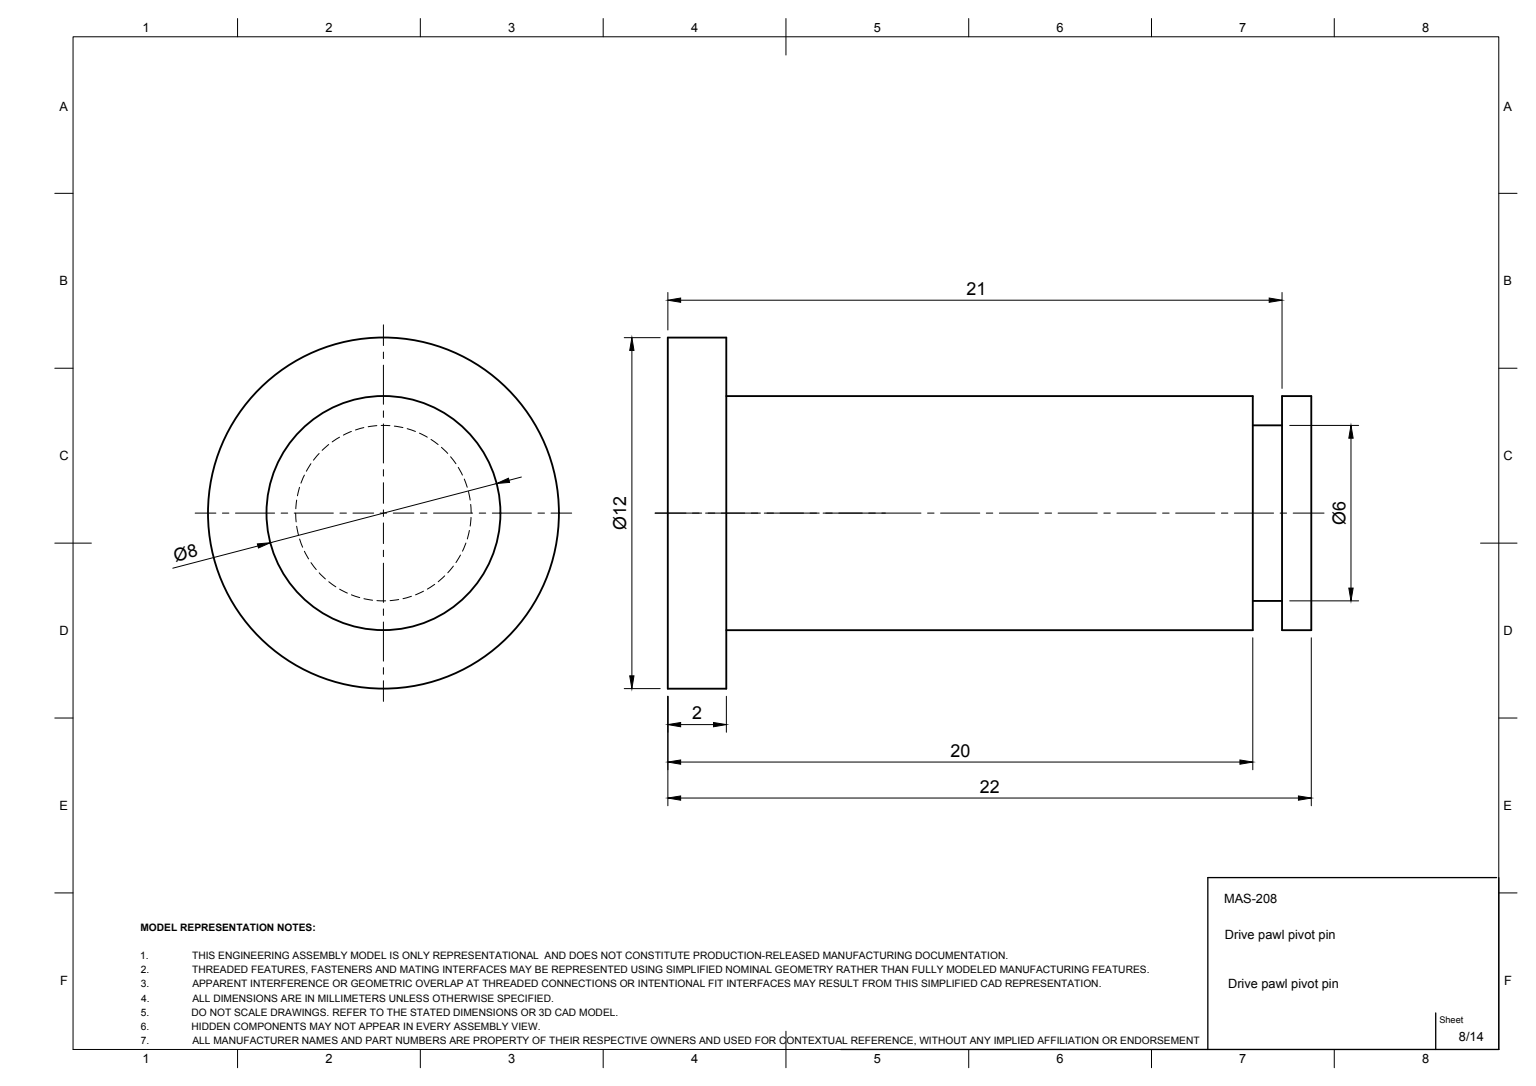
ISO-10303-21;
HEADER;
/* Generated by software containing ST-Developer
 * from STEP Tools, Inc. (www.steptools.com) 
 */

FILE_DESCRIPTION(
/* description */ ('Independent vertical20-tooth ratchet advance with repeated integral-c
ounterweight gravity pawls, swinging drive lever, bronze sleeves and f
ully retained axle stacks.18degpertooth. Native revolutes; geometric c
ycle checking rather than automatic contact/rolling dynamics. Gravity 
closing checked from actual pawl center of mass. Backplate/foot suppor
ts unit. Fits, torque, holding force, wear and life unassigned.'),
/* implementation_level */ '2;1');

FILE_NAME(
/* name */ 'Drive pawl pivot pin.step',
/* time_stamp */ '2026-11-09T06:25:53-08:00',
/* author */ (''),
/* organization */ (''),
/* preprocessor_version */ 'ST-DEVELOPER v20.2',
/* originating_system */ 'Autodesk Translation Framework v15.17.0.0',
/* authorisation */ '');

FILE_SCHEMA (('AUTOMOTIVE_DESIGN { 1 0 10303 214 3 1 1 }'));
ENDSEC;

DATA;
#10=MECHANICAL_DESIGN_GEOMETRIC_PRESENTATION_REPRESENTATION('',(#127),#4643);
#99=SHAPE_REPRESENTATION_RELATIONSHIP('SRR','None',#4704,#113);
#113=ADVANCED_BREP_SHAPE_REPRESENTATION('',(#141),#4633);
#127=STYLED_ITEM('',(#4782),#141);
#141=MANIFOLD_SOLID_BREP('Body1',#2663);
#174=FACE_BOUND('',#559,.T.);
#175=FACE_BOUND('',#561,.T.);
#176=FACE_BOUND('',#564,.T.);
#259=PLANE('',#2946);
#260=PLANE('',#2948);
#261=PLANE('',#2952);
#262=PLANE('',#2957);
#263=PLANE('',#2959);
#385=FACE_OUTER_BOUND('',#557,.T.);
#386=FACE_OUTER_BOUND('',#558,.T.);
#387=FACE_OUTER_BOUND('',#560,.T.);
#388=FACE_OUTER_BOUND('',#562,.T.);
#389=FACE_OUTER_BOUND('',#563,.T.);
#390=FACE_OUTER_BOUND('',#565,.T.);
#391=FACE_OUTER_BOUND('',#566,.T.);
#392=FACE_OUTER_BOUND('',#567,.T.);
#393=FACE_OUTER_BOUND('',#568,.T.);
#557=EDGE_LOOP('',(#2221,#2222,#2223,#2224));
#558=EDGE_LOOP('',(#2225));
#559=EDGE_LOOP('',(#2226));
#560=EDGE_LOOP('',(#2227));
#561=EDGE_LOOP('',(#2228));
#562=EDGE_LOOP('',(#2229,#2230,#2231,#2232));
#563=EDGE_LOOP('',(#2233));
#564=EDGE_LOOP('',(#2234));
#565=EDGE_LOOP('',(#2235,#2236,#2237,#2238));
#566=EDGE_LOOP('',(#2239));
#567=EDGE_LOOP('',(#2240,#2241,#2242,#2243));
#568=EDGE_LOOP('',(#2244));
#825=LINE('',#4308,#1087);
#826=LINE('',#4319,#1088);
#827=LINE('',#4327,#1089);
#828=LINE('',#4331,#1090);
#1087=VECTOR('',#3503,3.);
#1088=VECTOR('',#3518,4.);
#1089=VECTOR('',#3527,6.);
#1090=VECTOR('',#3534,4.);
#1195=CIRCLE('',#2944,3.);
#1196=CIRCLE('',#2945,3.);
#1197=CIRCLE('',#2947,4.);
#1198=CIRCLE('',#2949,4.);
#1199=CIRCLE('',#2951,4.);
#1200=CIRCLE('',#2953,6.);
#1201=CIRCLE('',#2954,4.);
#1202=CIRCLE('',#2956,6.);
#1381=VERTEX_POINT('',#4305);
#1382=VERTEX_POINT('',#4307);
#1383=VERTEX_POINT('',#4311);
#1384=VERTEX_POINT('',#4314);
#1385=VERTEX_POINT('',#4317);
#1386=VERTEX_POINT('',#4321);
#1387=VERTEX_POINT('',#4323);
#1388=VERTEX_POINT('',#4326);
#1675=EDGE_CURVE('',#1381,#1381,#1195,.T.);
#1676=EDGE_CURVE('',#1381,#1382,#825,.T.);
#1677=EDGE_CURVE('',#1382,#1382,#1196,.T.);
#1678=EDGE_CURVE('',#1383,#1383,#1197,.T.);
#1679=EDGE_CURVE('',#1384,#1384,#1198,.T.);
#1680=EDGE_CURVE('',#1385,#1385,#1199,.T.);
#1681=EDGE_CURVE('',#1385,#1384,#826,.T.);
#1682=EDGE_CURVE('',#1386,#1386,#1200,.T.);
#1683=EDGE_CURVE('',#1387,#1387,#1201,.T.);
#1684=EDGE_CURVE('',#1386,#1388,#827,.T.);
#1685=EDGE_CURVE('',#1388,#1388,#1202,.T.);
#1686=EDGE_CURVE('',#1383,#1387,#828,.T.);
#2221=ORIENTED_EDGE('',*,*,#1675,.T.);
#2222=ORIENTED_EDGE('',*,*,#1676,.T.);
#2223=ORIENTED_EDGE('',*,*,#1677,.F.);
#2224=ORIENTED_EDGE('',*,*,#1676,.F.);
#2225=ORIENTED_EDGE('',*,*,#1678,.F.);
#2226=ORIENTED_EDGE('',*,*,#1675,.F.);
#2227=ORIENTED_EDGE('',*,*,#1679,.F.);
#2228=ORIENTED_EDGE('',*,*,#1677,.T.);
#2229=ORIENTED_EDGE('',*,*,#1680,.F.);
#2230=ORIENTED_EDGE('',*,*,#1681,.T.);
#2231=ORIENTED_EDGE('',*,*,#1679,.T.);
#2232=ORIENTED_EDGE('',*,*,#1681,.F.);
#2233=ORIENTED_EDGE('',*,*,#1682,.T.);
#2234=ORIENTED_EDGE('',*,*,#1683,.F.);
#2235=ORIENTED_EDGE('',*,*,#1682,.F.);
#2236=ORIENTED_EDGE('',*,*,#1684,.T.);
#2237=ORIENTED_EDGE('',*,*,#1685,.T.);
#2238=ORIENTED_EDGE('',*,*,#1684,.F.);
#2239=ORIENTED_EDGE('',*,*,#1685,.F.);
#2240=ORIENTED_EDGE('',*,*,#1678,.T.);
#2241=ORIENTED_EDGE('',*,*,#1686,.T.);
#2242=ORIENTED_EDGE('',*,*,#1683,.T.);
#2243=ORIENTED_EDGE('',*,*,#1686,.F.);
#2244=ORIENTED_EDGE('',*,*,#1680,.T.);
#2487=CYLINDRICAL_SURFACE('',#2943,3.);
#2488=CYLINDRICAL_SURFACE('',#2950,4.);
#2489=CYLINDRICAL_SURFACE('',#2955,6.);
#2490=CYLINDRICAL_SURFACE('',#2958,4.);
#2591=ADVANCED_FACE('',(#385),#2487,.T.);
#2592=ADVANCED_FACE('',(#386,#174),#259,.F.);
#2593=ADVANCED_FACE('',(#387,#175),#260,.F.);
#2594=ADVANCED_FACE('',(#388),#2488,.T.);
#2595=ADVANCED_FACE('',(#389,#176),#261,.T.);
#2596=ADVANCED_FACE('',(#390),#2489,.T.);
#2597=ADVANCED_FACE('',(#391),#262,.F.);
#2598=ADVANCED_FACE('',(#392),#2490,.T.);
#2599=ADVANCED_FACE('',(#393),#263,.T.);
#2663=CLOSED_SHELL('',(#2591,#2592,#2593,#2594,#2595,#2596,#2597,#2598,
#2599));
#2942=AXIS2_PLACEMENT_3D('',#4303,#3497,#3498);
#2943=AXIS2_PLACEMENT_3D('',#4304,#3499,#3500);
#2944=AXIS2_PLACEMENT_3D('',#4306,#3501,#3502);
#2945=AXIS2_PLACEMENT_3D('',#4309,#3504,#3505);
#2946=AXIS2_PLACEMENT_3D('',#4310,#3506,#3507);
#2947=AXIS2_PLACEMENT_3D('',#4312,#3508,#3509);
#2948=AXIS2_PLACEMENT_3D('',#4313,#3510,#3511);
#2949=AXIS2_PLACEMENT_3D('',#4315,#3512,#3513);
#2950=AXIS2_PLACEMENT_3D('',#4316,#3514,#3515);
#2951=AXIS2_PLACEMENT_3D('',#4318,#3516,#3517);
#2952=AXIS2_PLACEMENT_3D('',#4320,#3519,#3520);
#2953=AXIS2_PLACEMENT_3D('',#4322,#3521,#3522);
#2954=AXIS2_PLACEMENT_3D('',#4324,#3523,#3524);
#2955=AXIS2_PLACEMENT_3D('',#4325,#3525,#3526);
#2956=AXIS2_PLACEMENT_3D('',#4328,#3528,#3529);
#2957=AXIS2_PLACEMENT_3D('',#4329,#3530,#3531);
#2958=AXIS2_PLACEMENT_3D('',#4330,#3532,#3533);
#2959=AXIS2_PLACEMENT_3D('',#4332,#3535,#3536);
#3497=DIRECTION('axis',(0.,0.,1.));
#3498=DIRECTION('refdir',(1.,0.,0.));
#3499=DIRECTION('center_axis',(0.,0.,1.));
#3500=DIRECTION('ref_axis',(1.,0.,0.));
#3501=DIRECTION('center_axis',(0.,0.,1.));
#3502=DIRECTION('ref_axis',(1.,0.,0.));
#3503=DIRECTION('',(0.,0.,1.));
#3504=DIRECTION('center_axis',(0.,0.,1.));
#3505=DIRECTION('ref_axis',(1.,0.,0.));
#3506=DIRECTION('center_axis',(0.,0.,-1.));
#3507=DIRECTION('ref_axis',(-1.,0.,0.));
#3508=DIRECTION('center_axis',(0.,0.,-1.));
#3509=DIRECTION('ref_axis',(1.,0.,0.));
#3510=DIRECTION('center_axis',(0.,0.,1.));
#3511=DIRECTION('ref_axis',(1.,0.,0.));
#3512=DIRECTION('center_axis',(0.,0.,1.));
#3513=DIRECTION('ref_axis',(1.,0.,0.));
#3514=DIRECTION('center_axis',(0.,0.,1.));
#3515=DIRECTION('ref_axis',(1.,0.,0.));
#3516=DIRECTION('center_axis',(0.,0.,1.));
#3517=DIRECTION('ref_axis',(1.,0.,0.));
#3518=DIRECTION('',(0.,0.,-1.));
#3519=DIRECTION('center_axis',(0.,0.,1.));
#3520=DIRECTION('ref_axis',(1.,0.,0.));
#3521=DIRECTION('center_axis',(0.,0.,1.));
#3522=DIRECTION('ref_axis',(1.,0.,0.));
#3523=DIRECTION('center_axis',(0.,0.,1.));
#3524=DIRECTION('ref_axis',(1.,0.,0.));
#3525=DIRECTION('center_axis',(0.,0.,1.));
#3526=DIRECTION('ref_axis',(1.,0.,0.));
#3527=DIRECTION('',(0.,0.,-1.));
#3528=DIRECTION('center_axis',(0.,0.,1.));
#3529=DIRECTION('ref_axis',(1.,0.,0.));
#3530=DIRECTION('center_axis',(0.,0.,1.));
#3531=DIRECTION('ref_axis',(1.,0.,0.));
#3532=DIRECTION('center_axis',(0.,0.,1.));
#3533=DIRECTION('ref_axis',(1.,0.,0.));
#3534=DIRECTION('',(0.,0.,-1.));
#3535=DIRECTION('center_axis',(0.,0.,1.));
#3536=DIRECTION('ref_axis',(1.,0.,0.));
#4303=CARTESIAN_POINT('',(0.,0.,0.));
#4304=CARTESIAN_POINT('Origin',(0.,0.,18.5));
#4305=CARTESIAN_POINT('',(-3.,-3.67394039744206E-16,18.));
#4306=CARTESIAN_POINT('Origin',(0.,0.,18.));
#4307=CARTESIAN_POINT('',(-3.,-3.67394039744206E-16,19.));
#4308=CARTESIAN_POINT('',(-3.,-3.67394039744206E-16,18.5));
#4309=CARTESIAN_POINT('Origin',(0.,0.,19.));
#4310=CARTESIAN_POINT('Origin',(7.,0.,18.));
#4311=CARTESIAN_POINT('',(-4.,4.89858719658941E-16,18.));
#4312=CARTESIAN_POINT('Origin',(0.,0.,18.));
#4313=CARTESIAN_POINT('Origin',(3.,0.,19.));
#4314=CARTESIAN_POINT('',(-4.,-4.89858719658941E-16,19.));
#4315=CARTESIAN_POINT('Origin',(0.,0.,19.));
#4316=CARTESIAN_POINT('Origin',(0.,0.,0.));
#4317=CARTESIAN_POINT('',(-4.,-4.89858719658941E-16,20.));
#4318=CARTESIAN_POINT('Origin',(0.,0.,20.));
#4319=CARTESIAN_POINT('',(-4.,-4.89858719658941E-16,0.));
#4320=CARTESIAN_POINT('Origin',(0.,0.,0.));
#4321=CARTESIAN_POINT('',(-6.,-7.34788079488412E-16,0.));
#4322=CARTESIAN_POINT('Origin',(0.,0.,0.));
#4323=CARTESIAN_POINT('',(-4.,-4.89858719658941E-16,0.));
#4324=CARTESIAN_POINT('Origin',(0.,0.,0.));
#4325=CARTESIAN_POINT('Origin',(0.,0.,-2.));
#4326=CARTESIAN_POINT('',(-6.,-7.34788079488412E-16,-2.));
#4327=CARTESIAN_POINT('',(-6.,-7.34788079488412E-16,-2.));
#4328=CARTESIAN_POINT('Origin',(0.,0.,-2.));
#4329=CARTESIAN_POINT('Origin',(0.,0.,-2.));
#4330=CARTESIAN_POINT('Origin',(0.,0.,0.));
#4331=CARTESIAN_POINT('',(-4.,-4.89858719658941E-16,0.));
#4332=CARTESIAN_POINT('Origin',(0.,0.,20.));
#4617=UNCERTAINTY_MEASURE_WITH_UNIT(LENGTH_MEASURE(0.01),#4644,
'DISTANCE_ACCURACY_VALUE',
'Maximum model space distance between geometric entities at asserted c
onnectivities');
#4627=UNCERTAINTY_MEASURE_WITH_UNIT(LENGTH_MEASURE(0.01),#4644,
'DISTANCE_ACCURACY_VALUE',
'Maximum model space distance between geometric entities at asserted c
onnectivities');
#4633=(
GEOMETRIC_REPRESENTATION_CONTEXT(3)
GLOBAL_UNCERTAINTY_ASSIGNED_CONTEXT((#4617))
GLOBAL_UNIT_ASSIGNED_CONTEXT((#4644,#4646,#4647))
REPRESENTATION_CONTEXT('','3D')
);
#4643=(
GEOMETRIC_REPRESENTATION_CONTEXT(3)
GLOBAL_UNCERTAINTY_ASSIGNED_CONTEXT((#4627))
GLOBAL_UNIT_ASSIGNED_CONTEXT((#4644,#4646,#4647))
REPRESENTATION_CONTEXT('','3D')
);
#4644=(
LENGTH_UNIT()
NAMED_UNIT(*)
SI_UNIT(.MILLI.,.METRE.)
);
#4646=(
NAMED_UNIT(*)
PLANE_ANGLE_UNIT()
SI_UNIT($,.RADIAN.)
);
#4647=(
NAMED_UNIT(*)
SI_UNIT($,.STERADIAN.)
SOLID_ANGLE_UNIT()
);
#4653=SHAPE_DEFINITION_REPRESENTATION(#4668,#4704);
#4668=PRODUCT_DEFINITION_SHAPE('',$,#4720);
#4704=SHAPE_REPRESENTATION('',(#2942),#4633);
#4714=PRODUCT_DEFINITION_CONTEXT('part definition',#4761,'design');
#4720=PRODUCT_DEFINITION('Drive pawl pivot pin','Drive pawl pivot pin',
#4735,#4714);
#4735=PRODUCT_DEFINITION_FORMATION('',$,#4768);
#4761=APPLICATION_CONTEXT(
'Core Data for Automotive Mechanical Design Process');
#4762=PRODUCT_CONTEXT('part definition',#4761,'mechanical');
#4768=PRODUCT('Drive pawl pivot pin','Drive pawl pivot pin',$,(#4762));
#4782=PRESENTATION_STYLE_ASSIGNMENT((#4791));
#4791=SURFACE_STYLE_USAGE(.BOTH.,#4800);
#4800=SURFACE_SIDE_STYLE('',(#4809));
#4809=SURFACE_STYLE_FILL_AREA(#4818);
#4818=FILL_AREA_STYLE('Axle gray',(#4827));
#4827=FILL_AREA_STYLE_COLOUR('Axle gray',#4836);
#4836=COLOUR_RGB('Axle gray',0.576470588235294,0.615686274509804,0.666666666666667);
ENDSEC;
END-ISO-10303-21;
